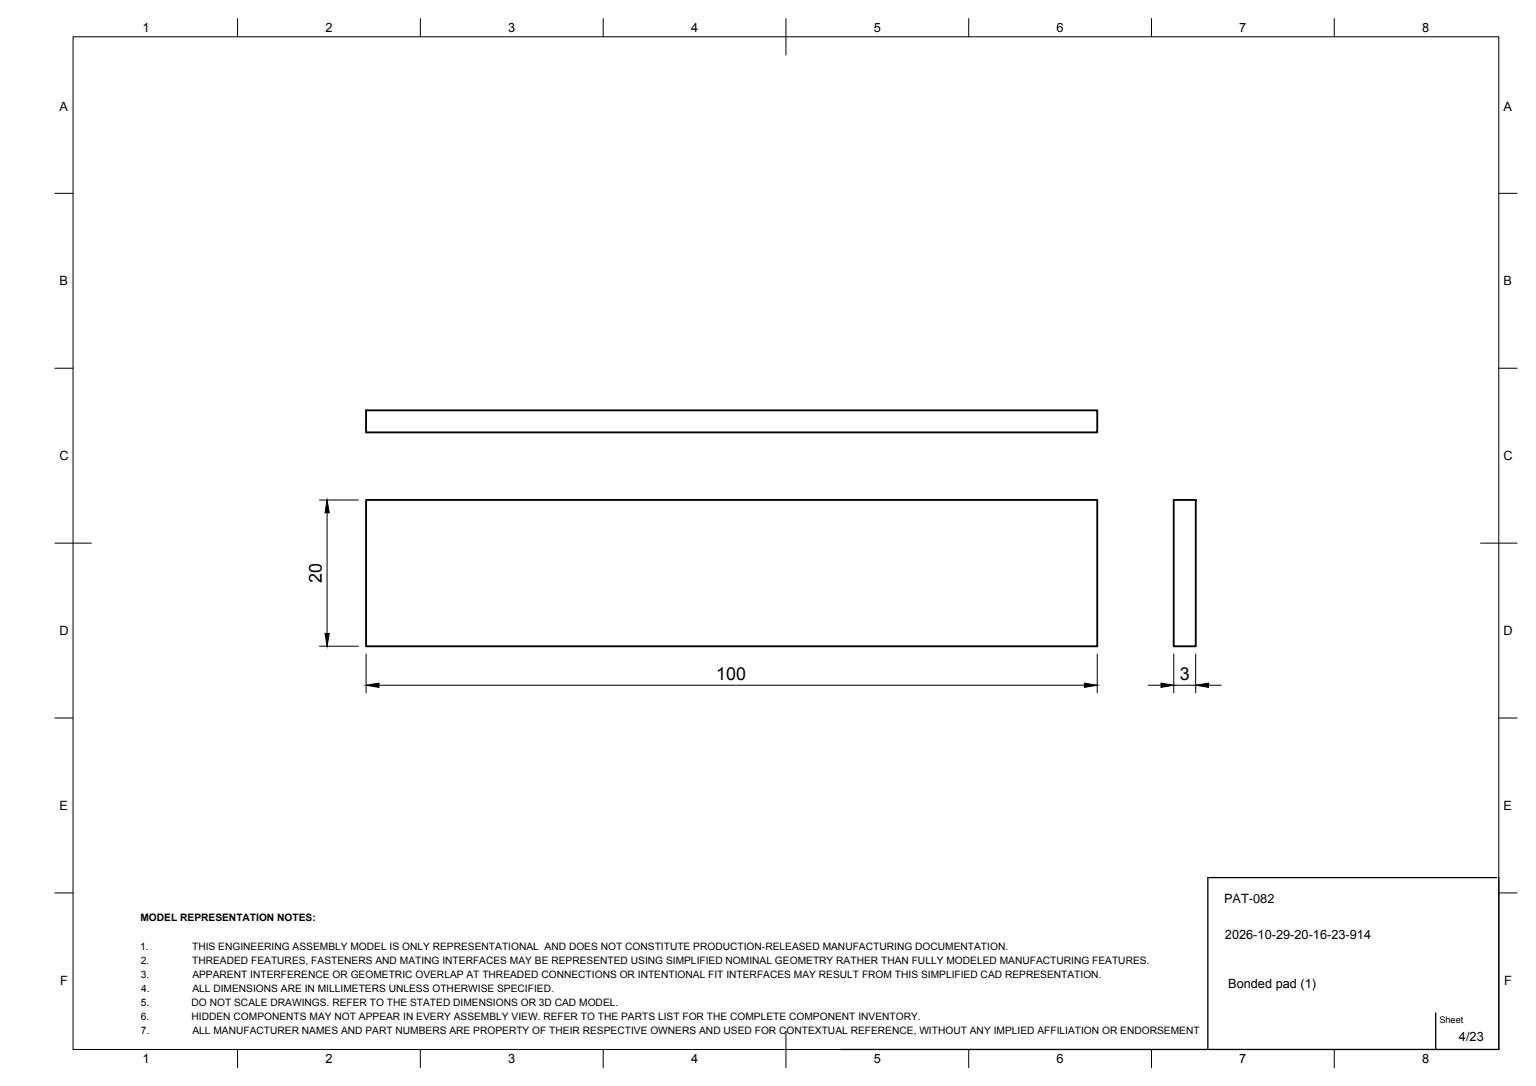
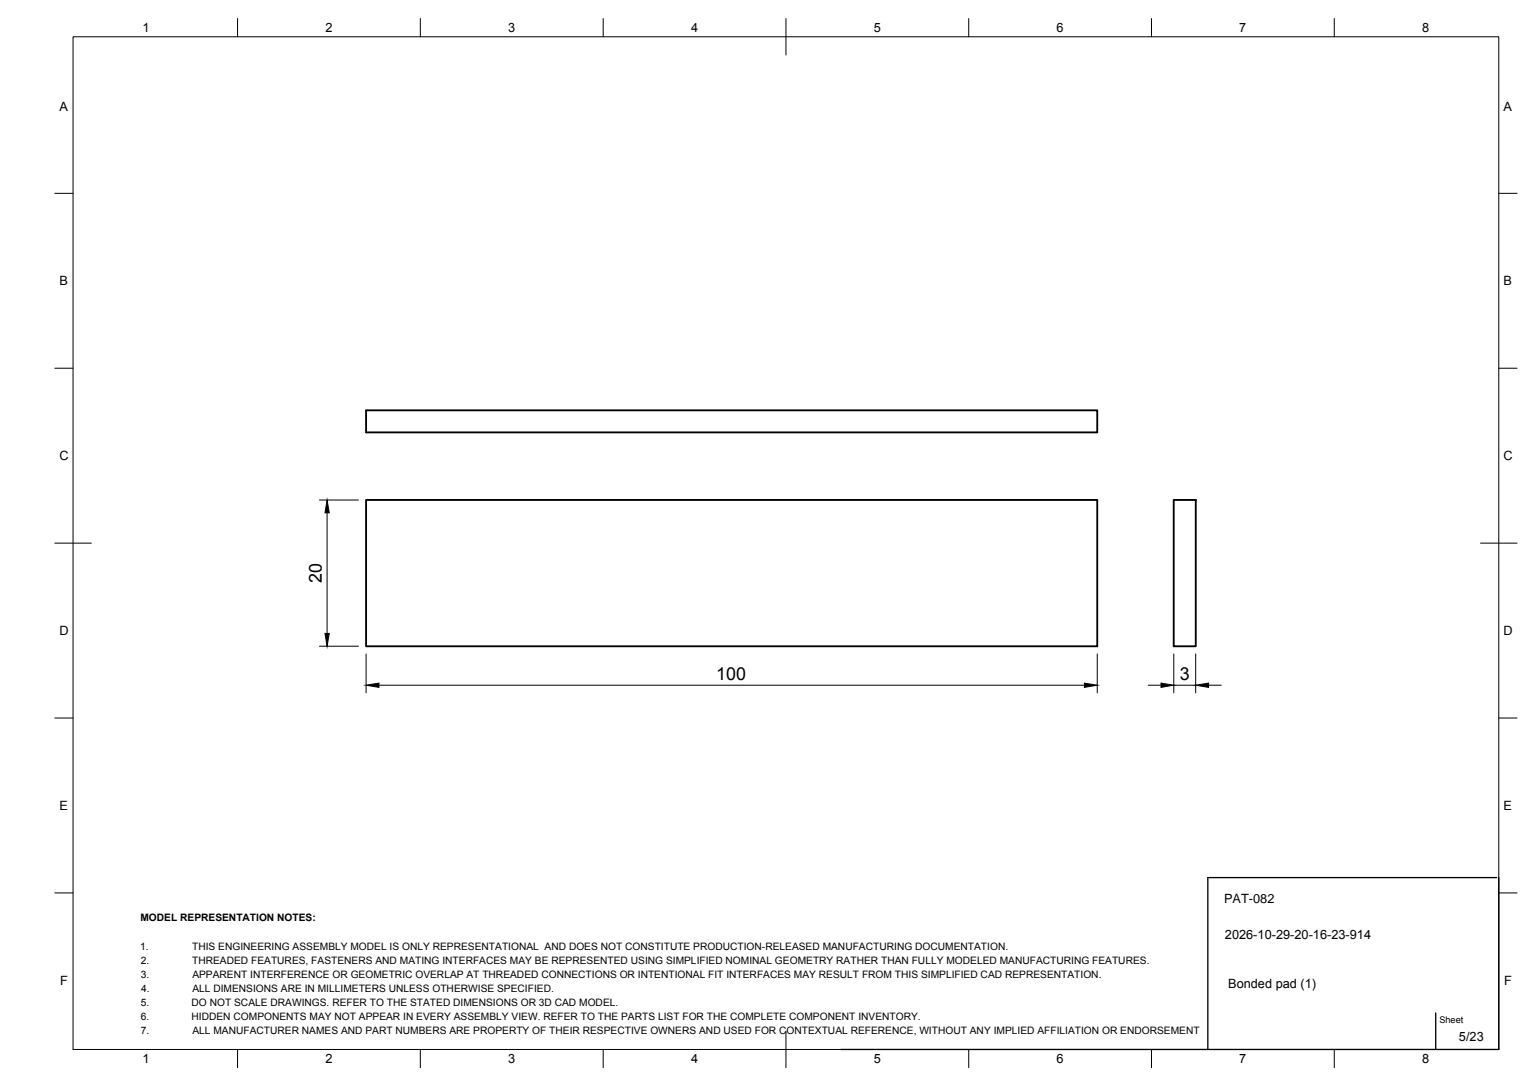
ISO-10303-21;
HEADER;
/* Generated by software containing ST-Developer
 * from STEP Tools, Inc. (www.steptools.com) 
 */

FILE_DESCRIPTION(
/* description */ ('PAT-082'),
/* implementation_level */ '2;1');

FILE_NAME(
/* name */ 'Bonded pad (1).step',
/* time_stamp */ '2026-10-29T20:16:13-07:00',
/* author */ (''),
/* organization */ (''),
/* preprocessor_version */ 'ST-DEVELOPER v20.2',
/* originating_system */ 'Autodesk Translation Framework v15.17.0.0',
/* authorisation */ '');

FILE_SCHEMA (('AUTOMOTIVE_DESIGN { 1 0 10303 214 3 1 1 }'));
ENDSEC;

DATA;
#10=MECHANICAL_DESIGN_GEOMETRIC_PRESENTATION_REPRESENTATION('',(#243),#8266);
#199=SHAPE_REPRESENTATION_RELATIONSHIP('SRR','None',#8361,#221);
#221=ADVANCED_BREP_SHAPE_REPRESENTATION('',(#265),#8245);
#243=STYLED_ITEM('',(#8551),#265);
#265=MANIFOLD_SOLID_BREP('Body1',#4583);
#421=PLANE('',#4893);
#422=PLANE('',#4894);
#423=PLANE('',#4895);
#424=PLANE('',#4896);
#425=PLANE('',#4897);
#426=PLANE('',#4898);
#596=FACE_OUTER_BOUND('',#878,.T.);
#597=FACE_OUTER_BOUND('',#879,.T.);
#598=FACE_OUTER_BOUND('',#880,.T.);
#599=FACE_OUTER_BOUND('',#881,.T.);
#600=FACE_OUTER_BOUND('',#882,.T.);
#601=FACE_OUTER_BOUND('',#883,.T.);
#878=EDGE_LOOP('',(#3182,#3183,#3184,#3185));
#879=EDGE_LOOP('',(#3186,#3187,#3188,#3189));
#880=EDGE_LOOP('',(#3190,#3191,#3192,#3193));
#881=EDGE_LOOP('',(#3194,#3195,#3196,#3197));
#882=EDGE_LOOP('',(#3198,#3199,#3200,#3201));
#883=EDGE_LOOP('',(#3202,#3203,#3204,#3205));
#1267=LINE('',#6914,#1622);
#1268=LINE('',#6916,#1623);
#1269=LINE('',#6918,#1624);
#1270=LINE('',#6919,#1625);
#1271=LINE('',#6922,#1626);
#1272=LINE('',#6924,#1627);
#1273=LINE('',#6925,#1628);
#1274=LINE('',#6928,#1629);
#1275=LINE('',#6930,#1630);
#1276=LINE('',#6931,#1631);
#1277=LINE('',#6933,#1632);
#1278=LINE('',#6934,#1633);
#1622=VECTOR('',#5504,1.);
#1623=VECTOR('',#5505,1.);
#1624=VECTOR('',#5506,1.);
#1625=VECTOR('',#5507,1.);
#1626=VECTOR('',#5510,1.);
#1627=VECTOR('',#5511,1.);
#1628=VECTOR('',#5512,1.);
#1629=VECTOR('',#5515,1.);
#1630=VECTOR('',#5516,1.);
#1631=VECTOR('',#5517,1.);
#1632=VECTOR('',#5520,1.);
#1633=VECTOR('',#5521,1.);
#2177=VERTEX_POINT('',#6912);
#2178=VERTEX_POINT('',#6913);
#2179=VERTEX_POINT('',#6915);
#2180=VERTEX_POINT('',#6917);
#2181=VERTEX_POINT('',#6921);
#2182=VERTEX_POINT('',#6923);
#2183=VERTEX_POINT('',#6927);
#2184=VERTEX_POINT('',#6929);
#2567=EDGE_CURVE('',#2177,#2178,#1267,.T.);
#2568=EDGE_CURVE('',#2178,#2179,#1268,.T.);
#2569=EDGE_CURVE('',#2180,#2179,#1269,.T.);
#2570=EDGE_CURVE('',#2177,#2180,#1270,.T.);
#2571=EDGE_CURVE('',#2181,#2177,#1271,.T.);
#2572=EDGE_CURVE('',#2182,#2180,#1272,.T.);
#2573=EDGE_CURVE('',#2181,#2182,#1273,.T.);
#2574=EDGE_CURVE('',#2183,#2181,#1274,.T.);
#2575=EDGE_CURVE('',#2184,#2182,#1275,.T.);
#2576=EDGE_CURVE('',#2183,#2184,#1276,.T.);
#2577=EDGE_CURVE('',#2178,#2183,#1277,.T.);
#2578=EDGE_CURVE('',#2179,#2184,#1278,.T.);
#3182=ORIENTED_EDGE('',*,*,#2567,.T.);
#3183=ORIENTED_EDGE('',*,*,#2568,.T.);
#3184=ORIENTED_EDGE('',*,*,#2569,.F.);
#3185=ORIENTED_EDGE('',*,*,#2570,.F.);
#3186=ORIENTED_EDGE('',*,*,#2571,.T.);
#3187=ORIENTED_EDGE('',*,*,#2570,.T.);
#3188=ORIENTED_EDGE('',*,*,#2572,.F.);
#3189=ORIENTED_EDGE('',*,*,#2573,.F.);
#3190=ORIENTED_EDGE('',*,*,#2574,.T.);
#3191=ORIENTED_EDGE('',*,*,#2573,.T.);
#3192=ORIENTED_EDGE('',*,*,#2575,.F.);
#3193=ORIENTED_EDGE('',*,*,#2576,.F.);
#3194=ORIENTED_EDGE('',*,*,#2577,.T.);
#3195=ORIENTED_EDGE('',*,*,#2576,.T.);
#3196=ORIENTED_EDGE('',*,*,#2578,.F.);
#3197=ORIENTED_EDGE('',*,*,#2568,.F.);
#3198=ORIENTED_EDGE('',*,*,#2578,.T.);
#3199=ORIENTED_EDGE('',*,*,#2575,.T.);
#3200=ORIENTED_EDGE('',*,*,#2572,.T.);
#3201=ORIENTED_EDGE('',*,*,#2569,.T.);
#3202=ORIENTED_EDGE('',*,*,#2577,.F.);
#3203=ORIENTED_EDGE('',*,*,#2567,.F.);
#3204=ORIENTED_EDGE('',*,*,#2571,.F.);
#3205=ORIENTED_EDGE('',*,*,#2574,.F.);
#4335=ADVANCED_FACE('',(#596),#421,.T.);
#4336=ADVANCED_FACE('',(#597),#422,.T.);
#4337=ADVANCED_FACE('',(#598),#423,.T.);
#4338=ADVANCED_FACE('',(#599),#424,.T.);
#4339=ADVANCED_FACE('',(#600),#425,.T.);
#4340=ADVANCED_FACE('',(#601),#426,.F.);
#4583=CLOSED_SHELL('',(#4335,#4336,#4337,#4338,#4339,#4340));
#4892=AXIS2_PLACEMENT_3D('',#6910,#5500,#5501);
#4893=AXIS2_PLACEMENT_3D('',#6911,#5502,#5503);
#4894=AXIS2_PLACEMENT_3D('',#6920,#5508,#5509);
#4895=AXIS2_PLACEMENT_3D('',#6926,#5513,#5514);
#4896=AXIS2_PLACEMENT_3D('',#6932,#5518,#5519);
#4897=AXIS2_PLACEMENT_3D('',#6935,#5522,#5523);
#4898=AXIS2_PLACEMENT_3D('',#6936,#5524,#5525);
#5500=DIRECTION('axis',(0.,0.,1.));
#5501=DIRECTION('refdir',(1.,0.,0.));
#5502=DIRECTION('center_axis',(0.,1.,0.));
#5503=DIRECTION('ref_axis',(-1.,0.,0.));
#5504=DIRECTION('',(-1.,0.,0.));
#5505=DIRECTION('',(0.,0.,1.));
#5506=DIRECTION('',(-1.,0.,0.));
#5507=DIRECTION('',(0.,0.,1.));
#5508=DIRECTION('center_axis',(1.,0.,0.));
#5509=DIRECTION('ref_axis',(0.,1.,0.));
#5510=DIRECTION('',(0.,1.,0.));
#5511=DIRECTION('',(0.,1.,0.));
#5512=DIRECTION('',(0.,0.,1.));
#5513=DIRECTION('center_axis',(0.,-1.,0.));
#5514=DIRECTION('ref_axis',(1.,0.,0.));
#5515=DIRECTION('',(1.,0.,0.));
#5516=DIRECTION('',(1.,0.,0.));
#5517=DIRECTION('',(0.,0.,1.));
#5518=DIRECTION('center_axis',(-1.,0.,0.));
#5519=DIRECTION('ref_axis',(0.,-1.,0.));
#5520=DIRECTION('',(0.,-1.,0.));
#5521=DIRECTION('',(0.,-1.,0.));
#5522=DIRECTION('center_axis',(0.,0.,1.));
#5523=DIRECTION('ref_axis',(1.,0.,0.));
#5524=DIRECTION('center_axis',(0.,0.,1.));
#5525=DIRECTION('ref_axis',(1.,0.,0.));
#6910=CARTESIAN_POINT('',(0.,0.,0.));
#6911=CARTESIAN_POINT('Origin',(8.,5.,-0.7));
#6912=CARTESIAN_POINT('',(8.,5.,-0.7));
#6913=CARTESIAN_POINT('',(6.,5.,-0.7));
#6914=CARTESIAN_POINT('',(8.,5.,-0.7));
#6915=CARTESIAN_POINT('',(6.,5.,-0.4));
#6916=CARTESIAN_POINT('',(6.,5.,-0.7));
#6917=CARTESIAN_POINT('',(8.,5.,-0.4));
#6918=CARTESIAN_POINT('',(8.,5.,-0.4));
#6919=CARTESIAN_POINT('',(8.,5.,-0.7));
#6920=CARTESIAN_POINT('Origin',(8.,-5.,-0.7));
#6921=CARTESIAN_POINT('',(8.,-5.,-0.7));
#6922=CARTESIAN_POINT('',(8.,-5.,-0.7));
#6923=CARTESIAN_POINT('',(8.,-5.,-0.4));
#6924=CARTESIAN_POINT('',(8.,-5.,-0.4));
#6925=CARTESIAN_POINT('',(8.,-5.,-0.7));
#6926=CARTESIAN_POINT('Origin',(6.,-5.,-0.7));
#6927=CARTESIAN_POINT('',(6.,-5.,-0.7));
#6928=CARTESIAN_POINT('',(6.,-5.,-0.7));
#6929=CARTESIAN_POINT('',(6.,-5.,-0.4));
#6930=CARTESIAN_POINT('',(6.,-5.,-0.4));
#6931=CARTESIAN_POINT('',(6.,-5.,-0.7));
#6932=CARTESIAN_POINT('Origin',(6.,5.,-0.7));
#6933=CARTESIAN_POINT('',(6.,5.,-0.7));
#6934=CARTESIAN_POINT('',(6.,5.,-0.4));
#6935=CARTESIAN_POINT('Origin',(7.,0.,-0.4));
#6936=CARTESIAN_POINT('Origin',(7.,0.,-0.7));
#8220=UNCERTAINTY_MEASURE_WITH_UNIT(LENGTH_MEASURE(0.001),#8267,
'DISTANCE_ACCURACY_VALUE',
'Maximum model space distance between geometric entities at asserted c
onnectivities');
#8241=UNCERTAINTY_MEASURE_WITH_UNIT(LENGTH_MEASURE(0.001),#8267,
'DISTANCE_ACCURACY_VALUE',
'Maximum model space distance between geometric entities at asserted c
onnectivities');
#8245=(
GEOMETRIC_REPRESENTATION_CONTEXT(3)
GLOBAL_UNCERTAINTY_ASSIGNED_CONTEXT((#8220))
GLOBAL_UNIT_ASSIGNED_CONTEXT((#8267,#8269,#8270))
REPRESENTATION_CONTEXT('','3D')
);
#8266=(
GEOMETRIC_REPRESENTATION_CONTEXT(3)
GLOBAL_UNCERTAINTY_ASSIGNED_CONTEXT((#8241))
GLOBAL_UNIT_ASSIGNED_CONTEXT((#8267,#8269,#8270))
REPRESENTATION_CONTEXT('','3D')
);
#8267=(
LENGTH_UNIT()
NAMED_UNIT(*)
SI_UNIT(.CENTI.,.METRE.)
);
#8269=(
NAMED_UNIT(*)
PLANE_ANGLE_UNIT()
SI_UNIT($,.RADIAN.)
);
#8270=(
NAMED_UNIT(*)
SI_UNIT($,.STERADIAN.)
SOLID_ANGLE_UNIT()
);
#8274=SHAPE_DEFINITION_REPRESENTATION(#8298,#8361);
#8298=PRODUCT_DEFINITION_SHAPE('',$,#8386);
#8361=SHAPE_REPRESENTATION('',(#4892),#8245);
#8382=PRODUCT_DEFINITION_CONTEXT('part definition',#8456,'design');
#8386=PRODUCT_DEFINITION('Bonded pad (1)','Bonded pad (1)',#8410,
#8382);
#8410=PRODUCT_DEFINITION_FORMATION('',$,#8461);
#8456=APPLICATION_CONTEXT(
'Core Data for Automotive Mechanical Design Process');
#8457=PRODUCT_CONTEXT('part definition',#8456,'mechanical');
#8461=PRODUCT('Bonded pad (1)','Bonded pad (1)','Bonded pad (1)',
(#8457));
#8545=COLOUR_RGB('Off White',0.89,0.88,0.83);
#8546=FILL_AREA_STYLE_COLOUR('',#8545);
#8547=FILL_AREA_STYLE('',(#8546));
#8548=SURFACE_STYLE_FILL_AREA(#8547);
#8549=SURFACE_SIDE_STYLE('',(#8548));
#8550=SURFACE_STYLE_USAGE(.BOTH.,#8549);
#8551=PRESENTATION_STYLE_ASSIGNMENT((#8550));
ENDSEC;
END-ISO-10303-21;
